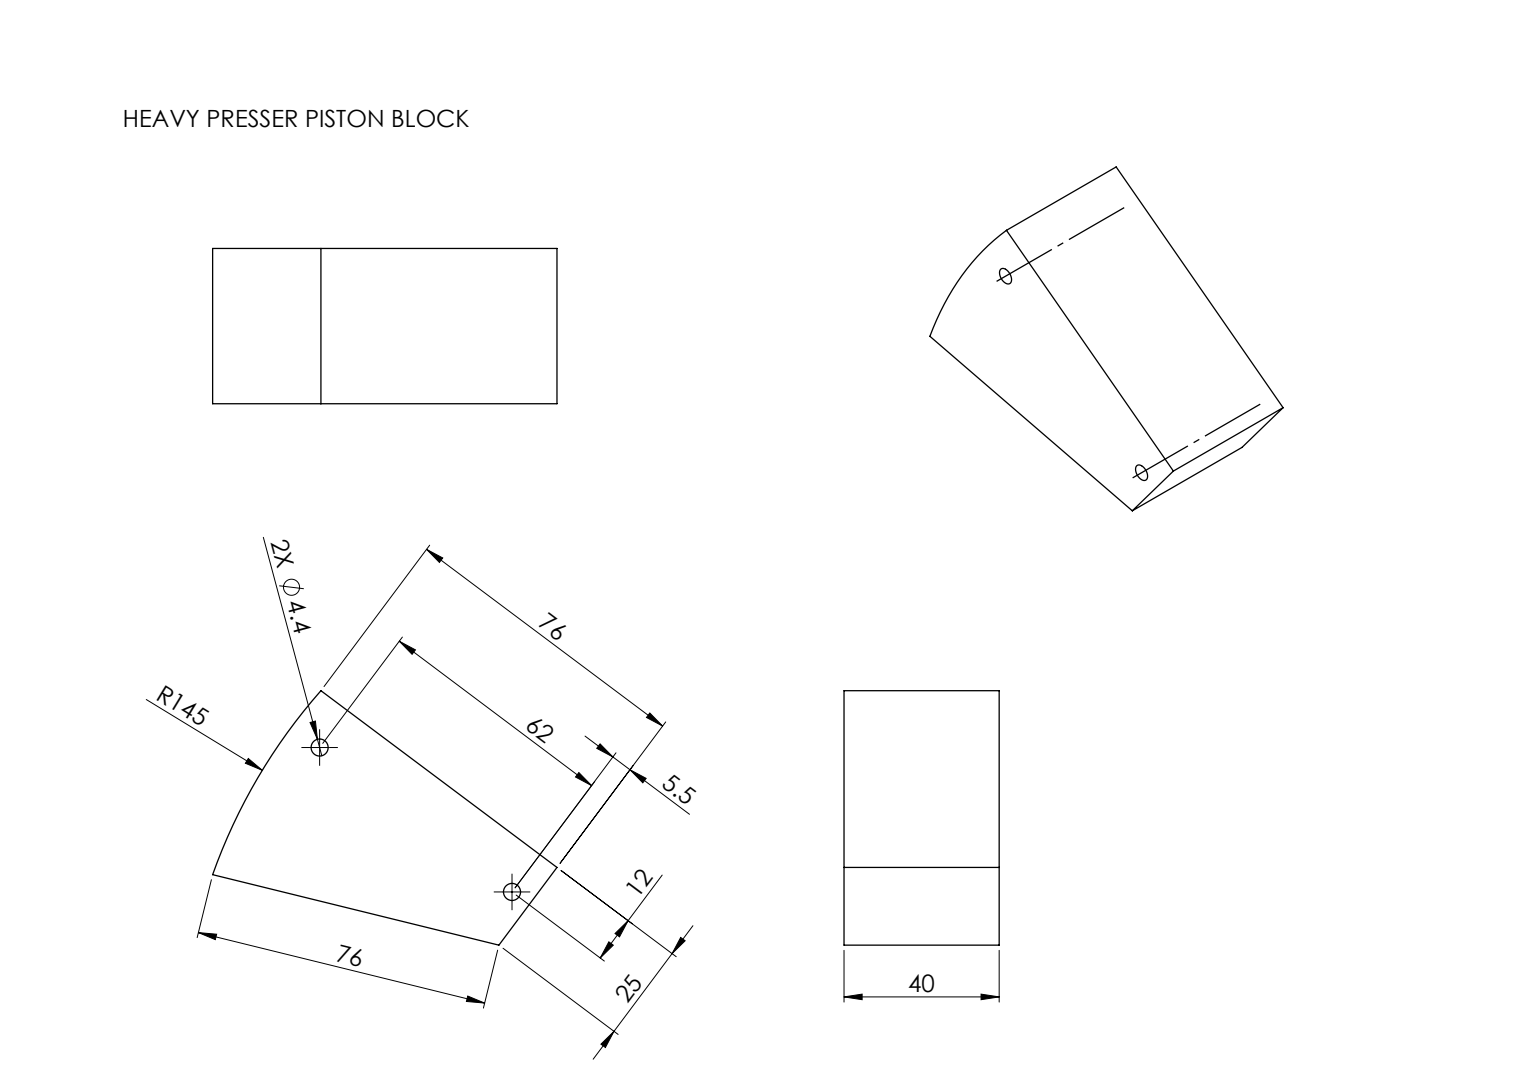
ISO-10303-21;
HEADER;
FILE_DESCRIPTION (('STEP AP214'),
    '1' );
FILE_NAME ('Heavy Presser Piston Block.step',
    '2026-10-02T13:02:33',
    ( '' ),
    ( '' ),
    'SwSTEP 2.0',
    'SolidWorks 2026',
    '' );
FILE_SCHEMA (( 'AUTOMOTIVE_DESIGN' ));
ENDSEC;

DATA;
#225=FACE_OUTER_BOUND ( 'NONE', #16348, .T. ) ;
#230=CIRCLE ( 'NONE', #18445, 2.199999999999993516 ) ;
#258=LINE ( 'NONE', #13329, #11510 ) ;
#263=CIRCLE ( 'NONE', #6336, 2.200000000000000178 ) ;
#304=EDGE_CURVE ( 'NONE', #7962, #8290, #17617, .T. ) ;
#354=ORIENTED_EDGE ( 'NONE', *, *, #5419, .T. ) ;
#480=LINE ( 'NONE', #6273, #9392 ) ;
#508=DIRECTION ( 'NONE',  ( 1.438274729681541867E-16, 6.252920376642369977E-17, -1.000000000000000000 ) ) ;
#603=VECTOR ( 'NONE', #5115, 1000.000000000000000 ) ;
#636=VECTOR ( 'NONE', #10205, 1000.000000000000000 ) ;
#682=DIRECTION ( 'NONE',  ( -0.5989998693185457634, -0.8007491221077704946, 0.000000000000000000 ) ) ;
#703=CARTESIAN_POINT ( 'NONE',  ( 11.59211860341528144, 6.314490184041265053, -130.3485206753969976 ) ) ;
#757=EDGE_CURVE ( 'NONE', #18512, #8290, #1358, .T. ) ;
#800=ORIENTED_EDGE ( 'NONE', *, *, #2006, .T. ) ;
#812=EDGE_CURVE ( 'NONE', #4040, #5969, #7036, .T. ) ;
#826=ORIENTED_EDGE ( 'NONE', *, *, #17274, .F. ) ;
#1048=DIRECTION ( 'NONE',  ( -8.693966348389027220E-17, 1.991237296706375196E-16, -1.000000000000000000 ) ) ;
#1092=AXIS2_PLACEMENT_3D ( 'NONE', #1303, #15296, #15670 ) ;
#1118=ORIENTED_EDGE ( 'NONE', *, *, #3119, .T. ) ;
#1303=CARTESIAN_POINT ( 'NONE',  ( 6.744699544032231168E-15, -6.824871242521816123E-15, 20.00000000000000000 ) ) ;
#1307=CARTESIAN_POINT ( 'NONE',  ( 59.44021041145193607, -44.12097743988038445, 19.99999999999998579 ) ) ;
#1317=FILL_AREA_STYLE ('',( #8512 ) ) ;
#1334=AXIS2_PLACEMENT_3D ( 'NONE', #11257, #3005, #8795 ) ;
#1340=CARTESIAN_POINT ( 'NONE',  ( 11.59211860341526723, 6.314490184041260612, -20.00000000000000355 ) ) ;
#1358=LINE ( 'NONE', #8913, #6063 ) ;
#1383=CARTESIAN_POINT ( 'NONE',  ( -49.59961335071797350, 39.40051552679457814, -130.3485206753969976 ) ) ;
#1474=( LENGTH_UNIT ( ) NAMED_UNIT ( * ) SI_UNIT ( .MILLI., .METRE. ) );
#1543=AXIS2_PLACEMENT_3D ( 'NONE', #3701, #15558, #2382 ) ;
#1556=VERTEX_POINT ( 'NONE', #2126 ) ;
#1587=CARTESIAN_POINT ( 'NONE',  ( -49.59961335071796640, 39.40051552679455682, -20.00000000000000355 ) ) ;
#1622=VERTEX_POINT ( 'NONE', #4870 ) ;
#1771=CARTESIAN_POINT ( 'NONE',  ( -3.382878129548352319, -13.70423786865302773, 19.99999999999999645 ) ) ;
#1801=CYLINDRICAL_SURFACE ( 'NONE', #9760, 145.0000000000000284 ) ;
#1818=ORIENTED_EDGE ( 'NONE', *, *, #4013, .F. ) ;
#1882=EDGE_CURVE ( 'NONE', #5969, #7962, #258, .T. ) ;
#1917=ORIENTED_EDGE ( 'NONE', *, *, #4374, .T. ) ;
#1927=DIRECTION ( 'NONE',  ( 8.693966348389027220E-17, -1.991237296706374949E-16, 1.000000000000000000 ) ) ;
#1934=CARTESIAN_POINT ( 'NONE',  ( -49.26481467677530190, 51.83848025225071865, -20.00000000000001421 ) ) ;
#2006=EDGE_CURVE ( 'NONE', #9635, #8612, #18574, .T. ) ;
#2126=CARTESIAN_POINT ( 'NONE',  ( 5.275328570166847961E-15, 2.200000000000001510, -20.00000000000000355 ) ) ;
#2227=SURFACE_STYLE_FILL_AREA ( #15211 ) ;
#2336=CARTESIAN_POINT ( 'NONE',  ( -49.59961335071795929, 37.20051552679455398, 20.00000000000001066 ) ) ;
#2382=DIRECTION ( 'NONE',  ( -1.000000000000000000, 0.000000000000000000, -1.435633221498047038E-16 ) ) ;
#2431=ADVANCED_FACE ( 'NONE', ( #3042 ), #14693, .F. ) ;
#2536=DIRECTION ( 'NONE',  ( -8.693966348389027220E-17, 1.991237296706375196E-16, -1.000000000000000000 ) ) ;
#2549=LINE ( 'NONE', #14757, #636 ) ;
#2593=UNCERTAINTY_MEASURE_WITH_UNIT (LENGTH_MEASURE( 1.000000000000000082E-05 ), #7823, 'distance_accuracy_value', 'NONE');
#2779=AXIS2_PLACEMENT_3D ( 'NONE', #14313, #5502, #12494 ) ;
#2849=ORIENTED_EDGE ( 'NONE', *, *, #304, .F. ) ;
#2864=EDGE_CURVE ( 'NONE', #1556, #9635, #3017, .T. ) ;
#2920=ORIENTED_EDGE ( 'NONE', *, *, #10157, .T. ) ;
#2956=SHAPE_DEFINITION_REPRESENTATION ( #3460, #10585 ) ;
#2963=CARTESIAN_POINT ( 'NONE',  ( -88.52719037593115559, 10.14639200037310296, -20.00000000000001066 ) ) ;
#3005=DIRECTION ( 'NONE',  ( 8.693966348389027220E-17, -1.991237296706374949E-16, 1.000000000000000000 ) ) ;
#3017=LINE ( 'NONE', #16196, #12595 ) ;
#3042=FACE_OUTER_BOUND ( 'NONE', #3280, .T. ) ;
#3119=EDGE_CURVE ( 'NONE', #5990, #11990, #7201, .T. ) ;
#3158=CIRCLE ( 'NONE', #1092, 2.200000000000000178 ) ;
#3167=ORIENTED_EDGE ( 'NONE', *, *, #11156, .T. ) ;
#3175=VERTEX_POINT ( 'NONE', #4231 ) ;
#3200=DIRECTION ( 'NONE',  ( 8.693966348389027220E-17, -1.991237296706374949E-16, 1.000000000000000000 ) ) ;
#3217=EDGE_LOOP ( 'NONE', ( #14505, #4465, #354, #5009 ) ) ;
#3226=( GEOMETRIC_REPRESENTATION_CONTEXT ( 3 ) GLOBAL_UNCERTAINTY_ASSIGNED_CONTEXT ( ( #4915 ) ) GLOBAL_UNIT_ASSIGNED_CONTEXT ( ( #1474, #15867, #11213 ) ) REPRESENTATION_CONTEXT ( 'NONE', 'WORKASPACE' ) );
#3280=EDGE_LOOP ( 'NONE', ( #13552, #18153, #3167, #1818 ) ) ;
#3334=CARTESIAN_POINT ( 'NONE',  ( -49.59961335071797350, 37.20051552679458240, -130.3485206753969976 ) ) ;
#3350=EDGE_CURVE ( 'NONE', #4040, #1622, #11071, .T. ) ;
#3460=PRODUCT_DEFINITION_SHAPE ( 'NONE', 'NONE',  #12765 ) ;
#3506=EDGE_LOOP ( 'NONE', ( #10567, #5841, #17066, #12591 ) ) ;
#3509=CYLINDRICAL_SURFACE ( 'NONE', #10443, 2.199999999999993516 ) ;
#3613=CIRCLE ( 'NONE', #13925, 145.0000000000000284 ) ;
#3701=CARTESIAN_POINT ( 'NONE',  ( 59.44021041145192896, -44.12097743988037735, -20.00000000000000355 ) ) ;
#3769=DIRECTION ( 'NONE',  ( -0.8007491221077704946, 0.5989998693185457634, 1.888919472620034684E-16 ) ) ;
#3772=ORIENTED_EDGE ( 'NONE', *, *, #3847, .T. ) ;
#3782=DIRECTION ( 'NONE',  ( -8.693966348389027220E-17, 1.991237296706375196E-16, -1.000000000000000000 ) ) ;
#3847=EDGE_CURVE ( 'NONE', #7962, #9877, #480, .T. ) ;
#3887=DIRECTION ( 'NONE',  ( -1.000000000000000000, 0.000000000000000000, 0.000000000000000000 ) ) ;
#3912=ORIENTED_EDGE ( 'NONE', *, *, #10157, .F. ) ;
#3966=CARTESIAN_POINT ( 'NONE',  ( 11.59211860341528144, 6.314490184041265053, -130.3485206753969976 ) ) ;
#4013=EDGE_CURVE ( 'NONE', #9877, #11838, #11025, .T. ) ;
#4040=VERTEX_POINT ( 'NONE', #1934 ) ;
#4091=PRODUCT_DEFINITION_CONTEXT ( 'detailed design', #8228, 'design' ) ;
#4209=DIRECTION ( 'NONE',  ( -8.693966348389027220E-17, 1.991237296706374949E-16, -1.000000000000000000 ) ) ;
#4231=CARTESIAN_POINT ( 'NONE',  ( 5.005906274354426217E-15, -2.199999999999998845, -20.00000000000000355 ) ) ;
#4237=ORIENTED_EDGE ( 'NONE', *, *, #13563, .T. ) ;
#4250=CYLINDRICAL_SURFACE ( 'NONE', #1334, 2.200000000000000178 ) ;
#4370=DIRECTION ( 'NONE',  ( -0.9710487832595061652, 0.2388812686885108671, 0.000000000000000000 ) ) ;
#4374=EDGE_CURVE ( 'NONE', #5969, #18512, #2549, .T. ) ;
#4391=VECTOR ( 'NONE', #13402, 1000.000000000000000 ) ;
#4419=VERTEX_POINT ( 'NONE', #1587 ) ;
#4465=ORIENTED_EDGE ( 'NONE', *, *, #3350, .T. ) ;
#4487=FACE_BOUND ( 'NONE', #12157, .T. ) ;
#4592=CARTESIAN_POINT ( 'NONE',  ( -3.382878129548365198, -13.70423786865299753, -130.3485206753969976 ) ) ;
#4695=ADVANCED_FACE ( 'NONE', ( #11107 ), #12825, .F. ) ;
#4843=VECTOR ( 'NONE', #11753, 1000.000000000000000 ) ;
#4849=EDGE_CURVE ( 'NONE', #1556, #3175, #7849, .T. ) ;
#4870=CARTESIAN_POINT ( 'NONE',  ( -49.26481467677529480, 51.83848025225069733, 20.00000000000001421 ) ) ;
#4915=UNCERTAINTY_MEASURE_WITH_UNIT (LENGTH_MEASURE( 1.000000000000000082E-05 ), #1474, 'distance_accuracy_value', 'NONE');
#5009=ORIENTED_EDGE ( 'NONE', *, *, #4374, .F. ) ;
#5115=DIRECTION ( 'NONE',  ( 8.693966348389027220E-17, -1.991237296706374949E-16, 1.000000000000000000 ) ) ;
#5268=ADVANCED_FACE ( 'NONE', ( #12203 ), #6554, .F. ) ;
#5382=CARTESIAN_POINT ( 'NONE',  ( -49.59961335071796640, 39.40051552679454971, 20.00000000000001066 ) ) ;
#5419=EDGE_CURVE ( 'NONE', #1622, #18512, #17553, .T. ) ;
#5425=DIRECTION ( 'NONE',  ( 0.000000000000000000, 1.000000000000000000, 1.914177628664062635E-16 ) ) ;
#5502=DIRECTION ( 'NONE',  ( 1.438274729681541867E-16, 6.252920376642369977E-17, -1.000000000000000000 ) ) ;
#5615=EDGE_CURVE ( 'NONE', #3175, #1556, #263, .T. ) ;
#5702=ORIENTED_EDGE ( 'NONE', *, *, #13651, .T. ) ;
#5718=DIRECTION ( 'NONE',  ( 1.438274729681541867E-16, 6.252920376642369977E-17, -1.000000000000000000 ) ) ;
#5737=DIRECTION ( 'NONE',  ( -0.9710487832595061652, 0.2388812686885108949, 1.369518533665900065E-16 ) ) ;
#5778=ORIENTED_EDGE ( 'NONE', *, *, #11895, .T. ) ;
#5816=DIRECTION ( 'NONE',  ( -0.5989998693185457634, -0.8007491221077703836, -1.387778780781445429E-16 ) ) ;
#5838=LINE ( 'NONE', #1383, #4843 ) ;
#5841=ORIENTED_EDGE ( 'NONE', *, *, #12541, .T. ) ;
#5960=DIRECTION ( 'NONE',  ( 0.8007491221077702725, -0.5989998693185459855, -1.826024711554533667E-16 ) ) ;
#5969=VERTEX_POINT ( 'NONE', #8459 ) ;
#5990=VERTEX_POINT ( 'NONE', #9959 ) ;
#6063=VECTOR ( 'NONE', #5816, 1000.000000000000114 ) ;
#6113=EDGE_LOOP ( 'NONE', ( #1118, #5778 ) ) ;
#6207=FACE_OUTER_BOUND ( 'NONE', #3217, .T. ) ;
#6234=AXIS2_PLACEMENT_3D ( 'NONE', #2963, #11488, #10265 ) ;
#6273=CARTESIAN_POINT ( 'NONE',  ( -77.18258565727084886, 4.450738551673815380, -20.00000000000000355 ) ) ;
#6291=ORIENTED_EDGE ( 'NONE', *, *, #4849, .T. ) ;
#6336=AXIS2_PLACEMENT_3D ( 'NONE', #10804, #508, #16441 ) ;
#6554=PLANE ( 'NONE',  #12638 ) ;
#6601=ORIENTED_EDGE ( 'NONE', *, *, #12754, .T. ) ;
#6619=AXIS2_PLACEMENT_3D ( 'NONE', #1307, #4209, #7090 ) ;
#6777=CARTESIAN_POINT ( 'NONE',  ( -49.59961335071796640, 37.20051552679456108, -20.00000000000000355 ) ) ;
#6798=CARTESIAN_POINT ( 'NONE',  ( -77.18258565727083464, 4.450738551673830479, -130.3485206753969976 ) ) ;
#6936=DIRECTION ( 'NONE',  ( 0.8007491221077702725, -0.5989998693185459855, 7.771473782954798134E-17 ) ) ;
#6985=PRODUCT_CONTEXT ( 'NONE', #9441, 'mechanical' ) ;
#7036=LINE ( 'NONE', #1340, #11176 ) ;
#7090=DIRECTION ( 'NONE',  ( 0.000000000000000000, 1.000000000000000000, 1.991237296706374949E-16 ) ) ;
#7103=SURFACE_STYLE_FILL_AREA ( #1317 ) ;
#7201=CIRCLE ( 'NONE', #8976, 2.199999999999993516 ) ;
#7473=DIRECTION ( 'NONE',  ( 0.000000000000000000, 0.000000000000000000, 1.000000000000000000 ) ) ;
#7629=CARTESIAN_POINT ( 'NONE',  ( -49.26481467677530901, 51.83848025225072575, -130.3485206753969976 ) ) ;
#7651=LINE ( 'NONE', #12059, #4391 ) ;
#7657=ORIENTED_EDGE ( 'NONE', *, *, #1882, .T. ) ;
#7711=ADVANCED_FACE ( 'NONE', ( #16488 ), #1801, .T. ) ;
#7715=DIRECTION ( 'NONE',  ( -0.5989998693185459855, -0.8007491221077702725, -1.073713046591392860E-16 ) ) ;
#7771=DIRECTION ( 'NONE',  ( 0.000000000000000000, -1.000000000000000000, 0.000000000000000000 ) ) ;
#7823=( LENGTH_UNIT ( ) NAMED_UNIT ( * ) SI_UNIT ( .MILLI., .METRE. ) );
#7849=CIRCLE ( 'NONE', #18496, 2.200000000000000178 ) ;
#7962=VERTEX_POINT ( 'NONE', #13628 ) ;
#8004=SURFACE_SIDE_STYLE ('',( #2227 ) ) ;
#8096=PRODUCT_DEFINITION_FORMATION_WITH_SPECIFIED_SOURCE ( 'ANY', '', #12080, .NOT_KNOWN. ) ;
#8228=APPLICATION_CONTEXT ( 'automotive_design' ) ;
#8233=CARTESIAN_POINT ( 'NONE',  ( -49.59961335071795929, 37.20051552679455398, 20.00000000000001066 ) ) ;
#8253=DIRECTION ( 'NONE',  ( 0.000000000000000000, -1.000000000000000000, 0.000000000000000000 ) ) ;
#8290=VERTEX_POINT ( 'NONE', #1771 ) ;
#8459=CARTESIAN_POINT ( 'NONE',  ( 11.59211860341529210, 6.314490184041242848, -20.00000000000000355 ) ) ;
#8495=FACE_BOUND ( 'NONE', #9874, .T. ) ;
#8497=DIRECTION ( 'NONE',  ( 8.693966348389027220E-17, -1.991237296706374949E-16, 1.000000000000000000 ) ) ;
#8512=FILL_AREA_STYLE_COLOUR ( '', #16896 ) ;
#8574=ORIENTED_EDGE ( 'NONE', *, *, #4849, .F. ) ;
#8612=VERTEX_POINT ( 'NONE', #9404 ) ;
#8773=( NAMED_UNIT ( * ) SI_UNIT ( $, .STERADIAN. ) SOLID_ANGLE_UNIT ( ) );
#8795=DIRECTION ( 'NONE',  ( 0.000000000000000000, -1.000000000000000000, 0.000000000000000000 ) ) ;
#8913=CARTESIAN_POINT ( 'NONE',  ( 11.59211860341529565, 6.314490184041233967, 20.00000000000000000 ) ) ;
#8976=AXIS2_PLACEMENT_3D ( 'NONE', #8233, #2536, #14001 ) ;
#9049=SHAPE_REPRESENTATION_RELATIONSHIP ( 'NONE' , 'NONE' ,  #10585, #16340 ) ;
#9177=CARTESIAN_POINT ( 'NONE',  ( -77.18258565727082043, 4.450738551673800281, 20.00000000000000711 ) ) ;
#9248=ADVANCED_FACE ( 'NONE', ( #12865 ), #4250, .F. ) ;
#9274=EDGE_LOOP ( 'NONE', ( #17022, #3912 ) ) ;
#9287=COLOUR_RGB ( '', 0.66274510, 0.83137255, 0.94901961) ;
#9308=PLANE ( 'NONE',  #12562 ) ;
#9320=EDGE_LOOP ( 'NONE', ( #10989, #1917, #13592, #2849 ) ) ;
#9392=VECTOR ( 'NONE', #10698, 1000.000000000000000 ) ;
#9404=CARTESIAN_POINT ( 'NONE',  ( 5.005906274354423851E-15, -2.200000000000007283, 20.00000000000000000 ) ) ;
#9434=FILL_AREA_STYLE_COLOUR ( '', #9287 ) ;
#9441=APPLICATION_CONTEXT ( 'automotive_design' ) ;
#9605=STYLED_ITEM ( 'NONE', ( #17621 ), #16340 ) ;
#9635=VERTEX_POINT ( 'NONE', #9824 ) ;
#9760=AXIS2_PLACEMENT_3D ( 'NONE', #17668, #3200, #14777 ) ;
#9781=ORIENTED_EDGE ( 'NONE', *, *, #12823, .F. ) ;
#9824=CARTESIAN_POINT ( 'NONE',  ( 5.275328570166844017E-15, 2.199999999999993072, 20.00000000000000000 ) ) ;
#9874=EDGE_LOOP ( 'NONE', ( #5702, #800 ) ) ;
#9877=VERTEX_POINT ( 'NONE', #18744 ) ;
#9959=CARTESIAN_POINT ( 'NONE',  ( -49.59961335071796640, 35.00051552679456535, 20.00000000000001066 ) ) ;
#9990=CIRCLE ( 'NONE', #1543, 145.0000000000000284 ) ;
#10074=CARTESIAN_POINT ( 'NONE',  ( -77.18258565727082043, 4.450738551673800281, 20.00000000000000711 ) ) ;
#10098=( LENGTH_UNIT ( ) NAMED_UNIT ( * ) SI_UNIT ( .MILLI., .METRE. ) );
#10133=ADVANCED_FACE ( 'NONE', ( #15720 ), #16799, .F. ) ;
#10157=EDGE_CURVE ( 'NONE', #4419, #16131, #11532, .T. ) ;
#10159=CARTESIAN_POINT ( 'NONE',  ( -49.59961335071797350, 37.20051552679458240, -130.3485206753969976 ) ) ;
#10164=PLANE ( 'NONE',  #6234 ) ;
#10205=DIRECTION ( 'NONE',  ( 8.693966348389027220E-17, -1.991237296706374949E-16, 1.000000000000000000 ) ) ;
#10241=DIRECTION ( 'NONE',  ( -1.000000000000000000, 0.000000000000000000, 0.000000000000000000 ) ) ;
#10265=DIRECTION ( 'NONE',  ( -0.7999937637212570785, 0.6000083149482993150, -7.754303923936027931E-17 ) ) ;
#10274=AXIS2_PLACEMENT_3D ( 'NONE', #10159, #13919, #7771 ) ;
#10422=CARTESIAN_POINT ( 'NONE',  ( -77.18258565727083464, 4.450738551673830479, -130.3485206753969976 ) ) ;
#10443=AXIS2_PLACEMENT_3D ( 'NONE', #3334, #1927, #12036 ) ;
#10498=ORIENTED_EDGE ( 'NONE', *, *, #5615, .F. ) ;
#10565=AXIS2_PLACEMENT_3D ( 'NONE', #2336, #1048, #17058 ) ;
#10567=ORIENTED_EDGE ( 'NONE', *, *, #18157, .T. ) ;
#10571=ORIENTED_EDGE ( 'NONE', *, *, #12541, .F. ) ;
#10585=SHAPE_REPRESENTATION ( 'Heavy Presser Piston Block', ( #18772 ), #17189 ) ;
#10698=DIRECTION ( 'NONE',  ( -0.9710487832595061652, 0.2388812686885108671, -1.247264370992099311E-16 ) ) ;
#10705=ORIENTED_EDGE ( 'NONE', *, *, #13651, .F. ) ;
#10804=CARTESIAN_POINT ( 'NONE',  ( 3.267113004676621661E-15, 1.140077944303684267E-15, -20.00000000000000355 ) ) ;
#10989=ORIENTED_EDGE ( 'NONE', *, *, #1882, .F. ) ;
#11025=LINE ( 'NONE', #6798, #12395 ) ;
#11071=LINE ( 'NONE', #7629, #14733 ) ;
#11097=DIRECTION ( 'NONE',  ( 1.438274729681541867E-16, 6.252920376642369977E-17, -1.000000000000000000 ) ) ;
#11107=FACE_OUTER_BOUND ( 'NONE', #11351, .T. ) ;
#11156=EDGE_CURVE ( 'NONE', #8290, #11838, #13008, .T. ) ;
#11159=DIRECTION ( 'NONE',  ( 8.693966348389027220E-17, -1.991237296706374949E-16, 1.000000000000000000 ) ) ;
#11176=VECTOR ( 'NONE', #6936, 1000.000000000000000 ) ;
#11213=( NAMED_UNIT ( * ) SI_UNIT ( $, .STERADIAN. ) SOLID_ANGLE_UNIT ( ) );
#11257=CARTESIAN_POINT ( 'NONE',  ( -6.326550248787502032E-15, 2.311308694482618949E-14, -130.3485206753969976 ) ) ;
#11351=EDGE_LOOP ( 'NONE', ( #10571, #2920, #4237, #18064 ) ) ;
#11411=SURFACE_STYLE_USAGE ( .BOTH. , #18689 ) ;
#11488=DIRECTION ( 'NONE',  ( 1.438274729681541621E-16, 6.252920376642371210E-17, -1.000000000000000000 ) ) ;
#11510=VECTOR ( 'NONE', #11886, 1000.000000000000000 ) ;
#11532=CIRCLE ( 'NONE', #2779, 2.199999999999993516 ) ;
#11563=CARTESIAN_POINT ( 'NONE',  ( 3.267113004676621661E-15, 1.140077944303684267E-15, -20.00000000000000355 ) ) ;
#11666=FACE_BOUND ( 'NONE', #6113, .T. ) ;
#11753=DIRECTION ( 'NONE',  ( 8.693966348389027220E-17, -1.991237296706374949E-16, 1.000000000000000000 ) ) ;
#11834=DIRECTION ( 'NONE',  ( 0.2388812686885108949, 0.9710487832595062763, 1.725905983023835105E-16 ) ) ;
#11838=VERTEX_POINT ( 'NONE', #9177 ) ;
#11886=DIRECTION ( 'NONE',  ( -0.5989998693185457634, -0.8007491221077704946, -1.362228425344026962E-16 ) ) ;
#11895=EDGE_CURVE ( 'NONE', #11990, #5990, #15420, .T. ) ;
#11990=VERTEX_POINT ( 'NONE', #5382 ) ;
#12036=DIRECTION ( 'NONE',  ( 0.000000000000000000, -1.000000000000000000, 0.000000000000000000 ) ) ;
#12059=CARTESIAN_POINT ( 'NONE',  ( -49.59961335071797350, 35.00051552679458666, -130.3485206753969976 ) ) ;
#12080=PRODUCT ( 'Heavy Presser Piston Block', 'Heavy Presser Piston Block', '', ( #6985 ) ) ;
#12157=EDGE_LOOP ( 'NONE', ( #10498, #8574 ) ) ;
#12203=FACE_OUTER_BOUND ( 'NONE', #9320, .T. ) ;
#12343=PRESENTATION_STYLE_ASSIGNMENT (( #13768 ) ) ;
#12395=VECTOR ( 'NONE', #8497, 1000.000000000000000 ) ;
#12494=DIRECTION ( 'NONE',  ( -1.000000000000000000, 0.000000000000000000, 0.000000000000000000 ) ) ;
#12541=EDGE_CURVE ( 'NONE', #4419, #11990, #5838, .T. ) ;
#12562=AXIS2_PLACEMENT_3D ( 'NONE', #703, #7715, #17784 ) ;
#12591=ORIENTED_EDGE ( 'NONE', *, *, #13563, .F. ) ;
#12595=VECTOR ( 'NONE', #17366, 1000.000000000000000 ) ;
#12638=AXIS2_PLACEMENT_3D ( 'NONE', #3966, #3769, #682 ) ;
#12660=CLOSED_SHELL ( 'NONE', ( #13944, #10133, #9248, #7711, #2431, #5268, #13994, #16576, #4695, #13886 ) ) ;
#12754=EDGE_CURVE ( 'NONE', #9877, #4040, #9990, .T. ) ;
#12765=PRODUCT_DEFINITION ( 'UNKNOWN', '', #8096, #4091 ) ;
#12823=EDGE_CURVE ( 'NONE', #11838, #1622, #3613, .T. ) ;
#12825=CYLINDRICAL_SURFACE ( 'NONE', #10274, 2.199999999999993516 ) ;
#12865=FACE_OUTER_BOUND ( 'NONE', #18123, .T. ) ;
#12913=FACE_BOUND ( 'NONE', #9274, .T. ) ;
#13008=LINE ( 'NONE', #10074, #17235 ) ;
#13148=CARTESIAN_POINT ( 'NONE',  ( 11.59211860341529565, 6.314490184041233967, 20.00000000000000000 ) ) ;
#13213=STYLED_ITEM ( 'NONE', ( #12343 ), #15126 ) ;
#13284=EDGE_LOOP ( 'NONE', ( #17557, #16829, #15153, #18721 ) ) ;
#13329=CARTESIAN_POINT ( 'NONE',  ( 11.59211860341528855, 6.314490184041240184, -20.00000000000000355 ) ) ;
#13402=DIRECTION ( 'NONE',  ( 8.693966348389027220E-17, -1.991237296706374949E-16, 1.000000000000000000 ) ) ;
#13552=ORIENTED_EDGE ( 'NONE', *, *, #3847, .F. ) ;
#13563=EDGE_CURVE ( 'NONE', #16131, #5990, #7651, .T. ) ;
#13592=ORIENTED_EDGE ( 'NONE', *, *, #757, .T. ) ;
#13611=CARTESIAN_POINT ( 'NONE',  ( 0.000000000000000000, 0.000000000000000000, 0.000000000000000000 ) ) ;
#13628=CARTESIAN_POINT ( 'NONE',  ( -3.382878129548355872, -13.70423786865302063, -19.99999999999998934 ) ) ;
#13651=EDGE_CURVE ( 'NONE', #8612, #9635, #3158, .T. ) ;
#13741=CARTESIAN_POINT ( 'NONE',  ( 59.44021041145193607, -44.12097743988038445, 19.99999999999998579 ) ) ;
#13768=SURFACE_STYLE_USAGE ( .BOTH. , #8004 ) ;
#13812=CARTESIAN_POINT ( 'NONE',  ( 11.59211860341529565, 6.314490184041233967, 20.00000000000000000 ) ) ;
#13886=ADVANCED_FACE ( 'NONE', ( #12913, #4487, #225 ), #10164, .T. ) ;
#13919=DIRECTION ( 'NONE',  ( 8.693966348389027220E-17, -1.991237296706374949E-16, 1.000000000000000000 ) ) ;
#13925=AXIS2_PLACEMENT_3D ( 'NONE', #13741, #3782, #5425 ) ;
#13944=ADVANCED_FACE ( 'NONE', ( #17976 ), #3509, .F. ) ;
#13994=ADVANCED_FACE ( 'NONE', ( #6207 ), #9308, .F. ) ;
#14001=DIRECTION ( 'NONE',  ( 0.000000000000000000, 1.000000000000000000, 0.000000000000000000 ) ) ;
#14149=MECHANICAL_DESIGN_GEOMETRIC_PRESENTATION_REPRESENTATION('',(#9605),#14495);
#14313=CARTESIAN_POINT ( 'NONE',  ( -49.59961335071796640, 37.20051552679456108, -20.00000000000000355 ) ) ;
#14417=EDGE_LOOP ( 'NONE', ( #17774, #14683, #10705, #826 ) ) ;
#14451=FACE_OUTER_BOUND ( 'NONE', #16321, .T. ) ;
#14495=( GEOMETRIC_REPRESENTATION_CONTEXT ( 3 ) GLOBAL_UNCERTAINTY_ASSIGNED_CONTEXT ( ( #2593 ) ) GLOBAL_UNIT_ASSIGNED_CONTEXT ( ( #7823, #16456, #16079 ) ) REPRESENTATION_CONTEXT ( 'NONE', 'WORKASPACE' ) );
#14505=ORIENTED_EDGE ( 'NONE', *, *, #812, .F. ) ;
#14622=ORIENTED_EDGE ( 'NONE', *, *, #5419, .F. ) ;
#14683=ORIENTED_EDGE ( 'NONE', *, *, #2864, .T. ) ;
#14693=PLANE ( 'NONE',  #15198 ) ;
#14713=ORIENTED_EDGE ( 'NONE', *, *, #757, .F. ) ;
#14731=DIRECTION ( 'NONE',  ( 8.693966348389027220E-17, -1.991237296706374949E-16, 1.000000000000000000 ) ) ;
#14733=VECTOR ( 'NONE', #16240, 1000.000000000000000 ) ;
#14757=CARTESIAN_POINT ( 'NONE',  ( 11.59211860341528144, 6.314490184041265053, -130.3485206753969976 ) ) ;
#14759=DIRECTION ( 'NONE',  ( 1.000000000000000000, 0.000000000000000000, 0.000000000000000000 ) ) ;
#14777=DIRECTION ( 'NONE',  ( 0.000000000000000000, -1.000000000000000000, -1.914177628664062635E-16 ) ) ;
#14807=VECTOR ( 'NONE', #5960, 1000.000000000000114 ) ;
#15126=MANIFOLD_SOLID_BREP ( 'Boss-Extrude1', #12660 ) ;
#15153=ORIENTED_EDGE ( 'NONE', *, *, #12823, .T. ) ;
#15178=AXIS2_PLACEMENT_3D ( 'NONE', #15445, #11159, #8253 ) ;
#15198=AXIS2_PLACEMENT_3D ( 'NONE', #10422, #11834, #4370 ) ;
#15211=FILL_AREA_STYLE ('',( #9434 ) ) ;
#15296=DIRECTION ( 'NONE',  ( -8.693966348389027220E-17, 1.991237296706375196E-16, -1.000000000000000000 ) ) ;
#15420=CIRCLE ( 'NONE', #10565, 2.199999999999993516 ) ;
#15445=CARTESIAN_POINT ( 'NONE',  ( -6.326550248787502032E-15, 2.311308694482618949E-14, -130.3485206753969976 ) ) ;
#15558=DIRECTION ( 'NONE',  ( 1.438274729681541867E-16, 6.252920376642369977E-17, -1.000000000000000000 ) ) ;
#15661=DIRECTION ( 'NONE',  ( -8.693966348389027220E-17, 1.991237296706375196E-16, -1.000000000000000000 ) ) ;
#15670=DIRECTION ( 'NONE',  ( 0.000000000000000000, 1.000000000000000000, 0.000000000000000000 ) ) ;
#15720=FACE_OUTER_BOUND ( 'NONE', #14417, .T. ) ;
#15814=CARTESIAN_POINT ( 'NONE',  ( -49.59961335071796640, 35.00051552679457245, -20.00000000000000355 ) ) ;
#15867=( NAMED_UNIT ( * ) PLANE_ANGLE_UNIT ( ) SI_UNIT ( $, .RADIAN. ) );
#15954=DIRECTION ( 'NONE',  ( 0.000000000000000000, 1.000000000000000000, 0.000000000000000000 ) ) ;
#16079=( NAMED_UNIT ( * ) SI_UNIT ( $, .STERADIAN. ) SOLID_ANGLE_UNIT ( ) );
#16131=VERTEX_POINT ( 'NONE', #15814 ) ;
#16133=ORIENTED_EDGE ( 'NONE', *, *, #2864, .F. ) ;
#16196=CARTESIAN_POINT ( 'NONE',  ( -6.057127952975085021E-15, 2.200000000000023270, -130.3485206753969976 ) ) ;
#16240=DIRECTION ( 'NONE',  ( 8.693966348389027220E-17, -1.991237296706374949E-16, 1.000000000000000000 ) ) ;
#16321=EDGE_LOOP ( 'NONE', ( #14622, #9781, #18742, #14713 ) ) ;
#16340=ADVANCED_BREP_SHAPE_REPRESENTATION ( '', ( #15126, #18772 ), #17189 ) ;
#16348=EDGE_LOOP ( 'NONE', ( #6601, #16848, #7657, #3772 ) ) ;
#16441=DIRECTION ( 'NONE',  ( -1.000000000000000000, 0.000000000000000000, 0.000000000000000000 ) ) ;
#16456=( NAMED_UNIT ( * ) PLANE_ANGLE_UNIT ( ) SI_UNIT ( $, .RADIAN. ) );
#16488=FACE_OUTER_BOUND ( 'NONE', #13284, .T. ) ;
#16576=ADVANCED_FACE ( 'NONE', ( #14451, #8495, #11666 ), #17501, .F. ) ;
#16599=LINE ( 'NONE', #16807, #603 ) ;
#16719=AXIS2_PLACEMENT_3D ( 'NONE', #18378, #15661, #15954 ) ;
#16799=CYLINDRICAL_SURFACE ( 'NONE', #15178, 2.200000000000000178 ) ;
#16807=CARTESIAN_POINT ( 'NONE',  ( -6.326550248787502032E-15, -2.199999999999977085, -130.3485206753969976 ) ) ;
#16829=ORIENTED_EDGE ( 'NONE', *, *, #4013, .T. ) ;
#16848=ORIENTED_EDGE ( 'NONE', *, *, #812, .T. ) ;
#16896=COLOUR_RGB ( '', 0.66274510, 0.83137255, 0.94901961) ;
#16958=VECTOR ( 'NONE', #14731, 1000.000000000000000 ) ;
#17022=ORIENTED_EDGE ( 'NONE', *, *, #18157, .F. ) ;
#17058=DIRECTION ( 'NONE',  ( 0.000000000000000000, 1.000000000000000000, 0.000000000000000000 ) ) ;
#17066=ORIENTED_EDGE ( 'NONE', *, *, #3119, .F. ) ;
#17189=( GEOMETRIC_REPRESENTATION_CONTEXT ( 3 ) GLOBAL_UNCERTAINTY_ASSIGNED_CONTEXT ( ( #18578 ) ) GLOBAL_UNIT_ASSIGNED_CONTEXT ( ( #10098, #17244, #8773 ) ) REPRESENTATION_CONTEXT ( 'NONE', 'WORKASPACE' ) );
#17235=VECTOR ( 'NONE', #5737, 1000.000000000000114 ) ;
#17244=( NAMED_UNIT ( * ) PLANE_ANGLE_UNIT ( ) SI_UNIT ( $, .RADIAN. ) );
#17274=EDGE_CURVE ( 'NONE', #3175, #8612, #16599, .T. ) ;
#17310=ORIENTED_EDGE ( 'NONE', *, *, #2006, .F. ) ;
#17366=DIRECTION ( 'NONE',  ( 8.693966348389027220E-17, -1.991237296706374949E-16, 1.000000000000000000 ) ) ;
#17501=PLANE ( 'NONE',  #6619 ) ;
#17553=LINE ( 'NONE', #13148, #14807 ) ;
#17557=ORIENTED_EDGE ( 'NONE', *, *, #12754, .F. ) ;
#17617=LINE ( 'NONE', #4592, #16958 ) ;
#17621=PRESENTATION_STYLE_ASSIGNMENT (( #11411 ) ) ;
#17668=CARTESIAN_POINT ( 'NONE',  ( 59.44021041145192186, -44.12097743988036314, -130.3485206753969976 ) ) ;
#17774=ORIENTED_EDGE ( 'NONE', *, *, #5615, .T. ) ;
#17784=DIRECTION ( 'NONE',  ( 0.8007491221077702725, -0.5989998693185459855, 0.000000000000000000 ) ) ;
#17976=FACE_OUTER_BOUND ( 'NONE', #3506, .T. ) ;
#18064=ORIENTED_EDGE ( 'NONE', *, *, #11895, .F. ) ;
#18104=MECHANICAL_DESIGN_GEOMETRIC_PRESENTATION_REPRESENTATION('',(#13213),#3226);
#18123=EDGE_LOOP ( 'NONE', ( #16133, #6291, #18204, #17310 ) ) ;
#18153=ORIENTED_EDGE ( 'NONE', *, *, #304, .T. ) ;
#18157=EDGE_CURVE ( 'NONE', #16131, #4419, #230, .T. ) ;
#18204=ORIENTED_EDGE ( 'NONE', *, *, #17274, .T. ) ;
#18378=CARTESIAN_POINT ( 'NONE',  ( 6.744699544032231168E-15, -6.824871242521816123E-15, 20.00000000000000000 ) ) ;
#18445=AXIS2_PLACEMENT_3D ( 'NONE', #6777, #11097, #3887 ) ;
#18496=AXIS2_PLACEMENT_3D ( 'NONE', #11563, #5718, #10241 ) ;
#18512=VERTEX_POINT ( 'NONE', #13812 ) ;
#18574=CIRCLE ( 'NONE', #16719, 2.200000000000000178 ) ;
#18578=UNCERTAINTY_MEASURE_WITH_UNIT (LENGTH_MEASURE( 1.000000000000000082E-05 ), #10098, 'distance_accuracy_value', 'NONE');
#18689=SURFACE_SIDE_STYLE ('',( #7103 ) ) ;
#18721=ORIENTED_EDGE ( 'NONE', *, *, #3350, .F. ) ;
#18742=ORIENTED_EDGE ( 'NONE', *, *, #11156, .F. ) ;
#18744=CARTESIAN_POINT ( 'NONE',  ( -77.18258565727082043, 4.450738551673809162, -20.00000000000001776 ) ) ;
#18772=AXIS2_PLACEMENT_3D ( 'NONE', #13611, #7473, #14759 ) ;
ENDSEC;
END-ISO-10303-21;
